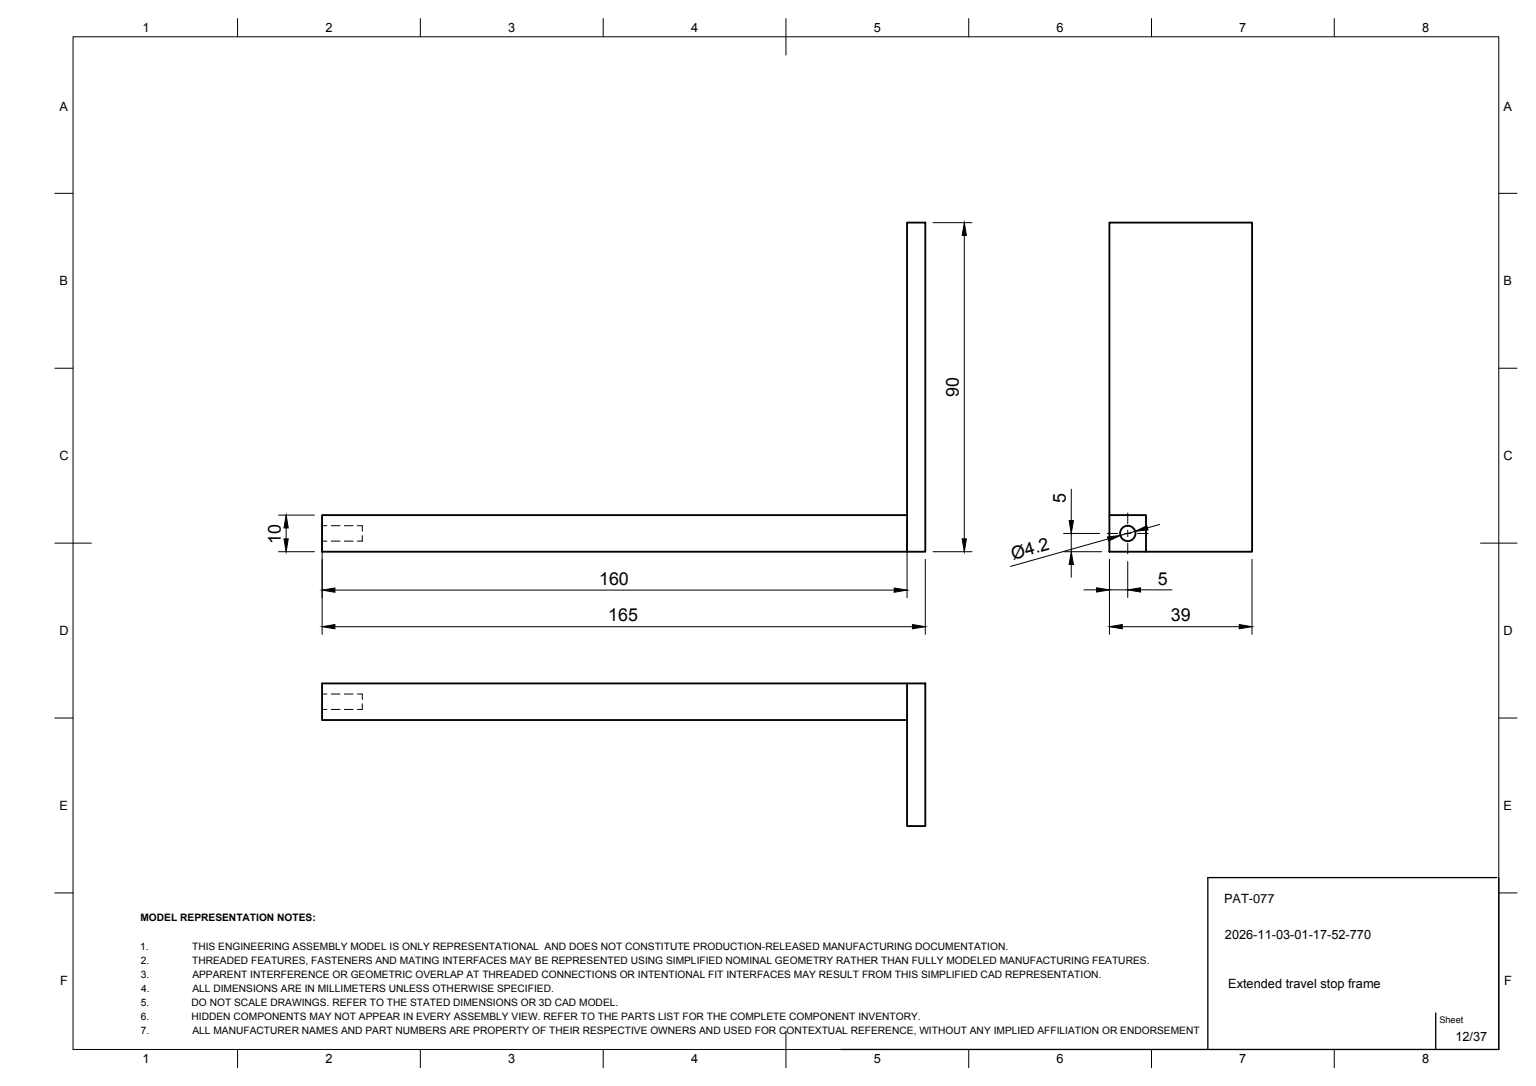
ISO-10303-21;
HEADER;
/* Generated by software containing ST-Developer
 * from STEP Tools, Inc. (www.steptools.com) 
 */

FILE_DESCRIPTION(
/* description */ ('Pallet stop with pneumatic fitting'),
/* implementation_level */ '2;1');

FILE_NAME(
/* name */ 'Extended travel stop frame.step',
/* time_stamp */ '2026-10-27T10:51:41-07:00',
/* author */ (''),
/* organization */ (''),
/* preprocessor_version */ 'ST-DEVELOPER v20.2',
/* originating_system */ 'Autodesk Translation Framework v15.17.0.0',
/* authorisation */ '');

FILE_SCHEMA (('AUTOMOTIVE_DESIGN { 1 0 10303 214 3 1 1 }'));
ENDSEC;

DATA;
#10=MECHANICAL_DESIGN_GEOMETRIC_PRESENTATION_REPRESENTATION('',(#364),#10265);
#300=SHAPE_REPRESENTATION_RELATIONSHIP('SRR','None',#10413,#332);
#332=ADVANCED_BREP_SHAPE_REPRESENTATION('',(#396),#10237);
#364=STYLED_ITEM('',(#10634),#396);
#396=MANIFOLD_SOLID_BREP('Body1',#5052);
#465=FACE_BOUND('',#1184,.T.);
#589=PLANE('',#5587);
#590=PLANE('',#5588);
#591=PLANE('',#5589);
#592=PLANE('',#5590);
#593=PLANE('',#5591);
#594=PLANE('',#5592);
#595=PLANE('',#5593);
#596=PLANE('',#5594);
#597=PLANE('',#5595);
#598=PLANE('',#5596);
#813=FACE_OUTER_BOUND('',#1173,.T.);
#814=FACE_OUTER_BOUND('',#1174,.T.);
#815=FACE_OUTER_BOUND('',#1175,.T.);
#816=FACE_OUTER_BOUND('',#1176,.T.);
#817=FACE_OUTER_BOUND('',#1177,.T.);
#818=FACE_OUTER_BOUND('',#1178,.T.);
#819=FACE_OUTER_BOUND('',#1179,.T.);
#820=FACE_OUTER_BOUND('',#1180,.T.);
#821=FACE_OUTER_BOUND('',#1181,.T.);
#822=FACE_OUTER_BOUND('',#1182,.T.);
#823=FACE_OUTER_BOUND('',#1183,.T.);
#1173=EDGE_LOOP('',(#3704,#3705,#3706,#3707));
#1174=EDGE_LOOP('',(#3708));
#1175=EDGE_LOOP('',(#3709,#3710,#3711,#3712,#3713,#3714));
#1176=EDGE_LOOP('',(#3715,#3716,#3717,#3718));
#1177=EDGE_LOOP('',(#3719,#3720,#3721,#3722));
#1178=EDGE_LOOP('',(#3723,#3724,#3725,#3726,#3727,#3728));
#1179=EDGE_LOOP('',(#3729,#3730,#3731,#3732,#3733,#3734));
#1180=EDGE_LOOP('',(#3735,#3736,#3737,#3738));
#1181=EDGE_LOOP('',(#3739,#3740,#3741,#3742));
#1182=EDGE_LOOP('',(#3743,#3744,#3745,#3746));
#1183=EDGE_LOOP('',(#3747,#3748,#3749,#3750));
#1184=EDGE_LOOP('',(#3751));
#1570=LINE('',#8908,#1905);
#1571=LINE('',#8914,#1906);
#1572=LINE('',#8916,#1907);
#1573=LINE('',#8918,#1908);
#1574=LINE('',#8920,#1909);
#1575=LINE('',#8922,#1910);
#1576=LINE('',#8923,#1911);
#1577=LINE('',#8926,#1912);
#1578=LINE('',#8928,#1913);
#1579=LINE('',#8929,#1914);
#1580=LINE('',#8932,#1915);
#1581=LINE('',#8933,#1916);
#1582=LINE('',#8937,#1917);
#1583=LINE('',#8939,#1918);
#1584=LINE('',#8940,#1919);
#1585=LINE('',#8941,#1920);
#1586=LINE('',#8944,#1921);
#1587=LINE('',#8945,#1922);
#1588=LINE('',#8946,#1923);
#1589=LINE('',#8949,#1924);
#1590=LINE('',#8950,#1925);
#1591=LINE('',#8952,#1926);
#1905=VECTOR('',#6477,0.21);
#1906=VECTOR('',#6484,1.);
#1907=VECTOR('',#6485,1.);
#1908=VECTOR('',#6486,1.);
#1909=VECTOR('',#6487,1.);
#1910=VECTOR('',#6488,1.);
#1911=VECTOR('',#6489,1.);
#1912=VECTOR('',#6492,1.);
#1913=VECTOR('',#6493,1.);
#1914=VECTOR('',#6494,1.);
#1915=VECTOR('',#6497,1.);
#1916=VECTOR('',#6498,1.);
#1917=VECTOR('',#6501,1.);
#1918=VECTOR('',#6502,1.);
#1919=VECTOR('',#6503,1.);
#1920=VECTOR('',#6504,1.);
#1921=VECTOR('',#6507,1.);
#1922=VECTOR('',#6508,1.);
#1923=VECTOR('',#6509,1.);
#1924=VECTOR('',#6512,1.);
#1925=VECTOR('',#6513,1.);
#1926=VECTOR('',#6516,1.);
#2226=CIRCLE('',#5585,0.21);
#2227=CIRCLE('',#5586,0.21);
#2505=VERTEX_POINT('',#8905);
#2506=VERTEX_POINT('',#8907);
#2507=VERTEX_POINT('',#8912);
#2508=VERTEX_POINT('',#8913);
#2509=VERTEX_POINT('',#8915);
#2510=VERTEX_POINT('',#8917);
#2511=VERTEX_POINT('',#8919);
#2512=VERTEX_POINT('',#8921);
#2513=VERTEX_POINT('',#8925);
#2514=VERTEX_POINT('',#8927);
#2515=VERTEX_POINT('',#8931);
#2516=VERTEX_POINT('',#8935);
#2517=VERTEX_POINT('',#8936);
#2518=VERTEX_POINT('',#8938);
#2519=VERTEX_POINT('',#8943);
#2520=VERTEX_POINT('',#8948);
#2951=EDGE_CURVE('',#2505,#2505,#2226,.T.);
#2952=EDGE_CURVE('',#2505,#2506,#1570,.T.);
#2953=EDGE_CURVE('',#2506,#2506,#2227,.T.);
#2954=EDGE_CURVE('',#2507,#2508,#1571,.T.);
#2955=EDGE_CURVE('',#2509,#2507,#1572,.T.);
#2956=EDGE_CURVE('',#2510,#2509,#1573,.T.);
#2957=EDGE_CURVE('',#2511,#2510,#1574,.T.);
#2958=EDGE_CURVE('',#2512,#2511,#1575,.T.);
#2959=EDGE_CURVE('',#2508,#2512,#1576,.T.);
#2960=EDGE_CURVE('',#2510,#2513,#1577,.T.);
#2961=EDGE_CURVE('',#2514,#2513,#1578,.T.);
#2962=EDGE_CURVE('',#2511,#2514,#1579,.T.);
#2963=EDGE_CURVE('',#2515,#2514,#1580,.T.);
#2964=EDGE_CURVE('',#2512,#2515,#1581,.T.);
#2965=EDGE_CURVE('',#2516,#2517,#1582,.T.);
#2966=EDGE_CURVE('',#2516,#2518,#1583,.T.);
#2967=EDGE_CURVE('',#2518,#2508,#1584,.T.);
#2968=EDGE_CURVE('',#2517,#2515,#1585,.T.);
#2969=EDGE_CURVE('',#2519,#2509,#1586,.T.);
#2970=EDGE_CURVE('',#2519,#2516,#1587,.T.);
#2971=EDGE_CURVE('',#2513,#2517,#1588,.T.);
#2972=EDGE_CURVE('',#2520,#2507,#1589,.T.);
#2973=EDGE_CURVE('',#2520,#2519,#1590,.T.);
#2974=EDGE_CURVE('',#2518,#2520,#1591,.T.);
#3704=ORIENTED_EDGE('',*,*,#2951,.F.);
#3705=ORIENTED_EDGE('',*,*,#2952,.T.);
#3706=ORIENTED_EDGE('',*,*,#2953,.T.);
#3707=ORIENTED_EDGE('',*,*,#2952,.F.);
#3708=ORIENTED_EDGE('',*,*,#2953,.F.);
#3709=ORIENTED_EDGE('',*,*,#2954,.F.);
#3710=ORIENTED_EDGE('',*,*,#2955,.F.);
#3711=ORIENTED_EDGE('',*,*,#2956,.F.);
#3712=ORIENTED_EDGE('',*,*,#2957,.F.);
#3713=ORIENTED_EDGE('',*,*,#2958,.F.);
#3714=ORIENTED_EDGE('',*,*,#2959,.F.);
#3715=ORIENTED_EDGE('',*,*,#2957,.T.);
#3716=ORIENTED_EDGE('',*,*,#2960,.T.);
#3717=ORIENTED_EDGE('',*,*,#2961,.F.);
#3718=ORIENTED_EDGE('',*,*,#2962,.F.);
#3719=ORIENTED_EDGE('',*,*,#2958,.T.);
#3720=ORIENTED_EDGE('',*,*,#2962,.T.);
#3721=ORIENTED_EDGE('',*,*,#2963,.F.);
#3722=ORIENTED_EDGE('',*,*,#2964,.F.);
#3723=ORIENTED_EDGE('',*,*,#2965,.F.);
#3724=ORIENTED_EDGE('',*,*,#2966,.T.);
#3725=ORIENTED_EDGE('',*,*,#2967,.T.);
#3726=ORIENTED_EDGE('',*,*,#2959,.T.);
#3727=ORIENTED_EDGE('',*,*,#2964,.T.);
#3728=ORIENTED_EDGE('',*,*,#2968,.F.);
#3729=ORIENTED_EDGE('',*,*,#2969,.F.);
#3730=ORIENTED_EDGE('',*,*,#2970,.T.);
#3731=ORIENTED_EDGE('',*,*,#2965,.T.);
#3732=ORIENTED_EDGE('',*,*,#2971,.F.);
#3733=ORIENTED_EDGE('',*,*,#2960,.F.);
#3734=ORIENTED_EDGE('',*,*,#2956,.T.);
#3735=ORIENTED_EDGE('',*,*,#2955,.T.);
#3736=ORIENTED_EDGE('',*,*,#2972,.F.);
#3737=ORIENTED_EDGE('',*,*,#2973,.T.);
#3738=ORIENTED_EDGE('',*,*,#2969,.T.);
#3739=ORIENTED_EDGE('',*,*,#2954,.T.);
#3740=ORIENTED_EDGE('',*,*,#2967,.F.);
#3741=ORIENTED_EDGE('',*,*,#2974,.T.);
#3742=ORIENTED_EDGE('',*,*,#2972,.T.);
#3743=ORIENTED_EDGE('',*,*,#2971,.T.);
#3744=ORIENTED_EDGE('',*,*,#2968,.T.);
#3745=ORIENTED_EDGE('',*,*,#2963,.T.);
#3746=ORIENTED_EDGE('',*,*,#2961,.T.);
#3747=ORIENTED_EDGE('',*,*,#2970,.F.);
#3748=ORIENTED_EDGE('',*,*,#2973,.F.);
#3749=ORIENTED_EDGE('',*,*,#2974,.F.);
#3750=ORIENTED_EDGE('',*,*,#2966,.F.);
#3751=ORIENTED_EDGE('',*,*,#2951,.T.);
#4654=CYLINDRICAL_SURFACE('',#5584,0.21);
#4808=ADVANCED_FACE('',(#813),#4654,.F.);
#4809=ADVANCED_FACE('',(#814),#589,.F.);
#4810=ADVANCED_FACE('',(#815),#590,.F.);
#4811=ADVANCED_FACE('',(#816),#591,.T.);
#4812=ADVANCED_FACE('',(#817),#592,.T.);
#4813=ADVANCED_FACE('',(#818),#593,.T.);
#4814=ADVANCED_FACE('',(#819),#594,.T.);
#4815=ADVANCED_FACE('',(#820),#595,.T.);
#4816=ADVANCED_FACE('',(#821),#596,.T.);
#4817=ADVANCED_FACE('',(#822),#597,.T.);
#4818=ADVANCED_FACE('',(#823,#465),#598,.F.);
#5052=CLOSED_SHELL('',(#4808,#4809,#4810,#4811,#4812,#4813,#4814,#4815,
#4816,#4817,#4818));
#5583=AXIS2_PLACEMENT_3D('',#8903,#6471,#6472);
#5584=AXIS2_PLACEMENT_3D('',#8904,#6473,#6474);
#5585=AXIS2_PLACEMENT_3D('',#8906,#6475,#6476);
#5586=AXIS2_PLACEMENT_3D('',#8909,#6478,#6479);
#5587=AXIS2_PLACEMENT_3D('',#8910,#6480,#6481);
#5588=AXIS2_PLACEMENT_3D('',#8911,#6482,#6483);
#5589=AXIS2_PLACEMENT_3D('',#8924,#6490,#6491);
#5590=AXIS2_PLACEMENT_3D('',#8930,#6495,#6496);
#5591=AXIS2_PLACEMENT_3D('',#8934,#6499,#6500);
#5592=AXIS2_PLACEMENT_3D('',#8942,#6505,#6506);
#5593=AXIS2_PLACEMENT_3D('',#8947,#6510,#6511);
#5594=AXIS2_PLACEMENT_3D('',#8951,#6514,#6515);
#5595=AXIS2_PLACEMENT_3D('',#8953,#6517,#6518);
#5596=AXIS2_PLACEMENT_3D('',#8954,#6519,#6520);
#6471=DIRECTION('axis',(0.,0.,1.));
#6472=DIRECTION('refdir',(1.,0.,0.));
#6473=DIRECTION('center_axis',(0.,0.,1.));
#6474=DIRECTION('ref_axis',(1.,0.,0.));
#6475=DIRECTION('center_axis',(0.,0.,1.));
#6476=DIRECTION('ref_axis',(1.,0.,0.));
#6477=DIRECTION('',(0.,0.,1.));
#6478=DIRECTION('center_axis',(0.,0.,1.));
#6479=DIRECTION('ref_axis',(1.,0.,0.));
#6480=DIRECTION('center_axis',(0.,0.,1.));
#6481=DIRECTION('ref_axis',(1.,0.,0.));
#6482=DIRECTION('center_axis',(0.,0.,1.));
#6483=DIRECTION('ref_axis',(1.,0.,0.));
#6484=DIRECTION('',(0.,-1.,0.));
#6485=DIRECTION('',(1.,0.,0.));
#6486=DIRECTION('',(0.,-1.,0.));
#6487=DIRECTION('',(-1.,0.,0.));
#6488=DIRECTION('',(0.,1.,0.));
#6489=DIRECTION('',(1.,0.,0.));
#6490=DIRECTION('center_axis',(0.,1.,0.));
#6491=DIRECTION('ref_axis',(-1.,0.,0.));
#6492=DIRECTION('',(0.,0.,1.));
#6493=DIRECTION('',(-1.,0.,0.));
#6494=DIRECTION('',(0.,0.,1.));
#6495=DIRECTION('center_axis',(1.,0.,0.));
#6496=DIRECTION('ref_axis',(0.,1.,0.));
#6497=DIRECTION('',(0.,1.,0.));
#6498=DIRECTION('',(0.,0.,1.));
#6499=DIRECTION('center_axis',(0.,-1.,0.));
#6500=DIRECTION('ref_axis',(1.,0.,0.));
#6501=DIRECTION('',(0.,0.,1.));
#6502=DIRECTION('',(1.,0.,0.));
#6503=DIRECTION('',(0.,0.,1.));
#6504=DIRECTION('',(1.,0.,0.));
#6505=DIRECTION('center_axis',(-1.,0.,0.));
#6506=DIRECTION('ref_axis',(0.,-1.,0.));
#6507=DIRECTION('',(0.,0.,1.));
#6508=DIRECTION('',(0.,-1.,0.));
#6509=DIRECTION('',(0.,-1.,0.));
#6510=DIRECTION('center_axis',(0.,1.,0.));
#6511=DIRECTION('ref_axis',(-1.,0.,0.));
#6512=DIRECTION('',(0.,0.,1.));
#6513=DIRECTION('',(-1.,0.,0.));
#6514=DIRECTION('center_axis',(1.,0.,0.));
#6515=DIRECTION('ref_axis',(0.,1.,0.));
#6516=DIRECTION('',(0.,1.,0.));
#6517=DIRECTION('center_axis',(0.,0.,1.));
#6518=DIRECTION('ref_axis',(1.,0.,0.));
#6519=DIRECTION('center_axis',(0.,0.,1.));
#6520=DIRECTION('ref_axis',(1.,0.,0.));
#8903=CARTESIAN_POINT('',(0.,0.,0.));
#8904=CARTESIAN_POINT('Origin',(-4.,-3.,-0.1));
#8905=CARTESIAN_POINT('',(-4.21,-3.,0.));
#8906=CARTESIAN_POINT('Origin',(-4.,-3.,0.));
#8907=CARTESIAN_POINT('',(-4.21,-3.,1.1));
#8908=CARTESIAN_POINT('',(-4.21,-3.,-0.1));
#8909=CARTESIAN_POINT('Origin',(-4.,-3.,1.1));
#8910=CARTESIAN_POINT('Origin',(-4.,-3.,1.1));
#8911=CARTESIAN_POINT('Origin',(0.,-1.55,16.));
#8912=CARTESIAN_POINT('',(-3.5,-2.5,16.));
#8913=CARTESIAN_POINT('',(-3.5,-3.5,16.));
#8914=CARTESIAN_POINT('',(-3.5,-2.525,16.));
#8915=CARTESIAN_POINT('',(-4.5,-2.5,16.));
#8916=CARTESIAN_POINT('',(-1.75,-2.5,16.));
#8917=CARTESIAN_POINT('',(-4.5,0.4,16.));
#8918=CARTESIAN_POINT('',(-4.5,0.4,16.));
#8919=CARTESIAN_POINT('',(4.5,0.4,16.));
#8920=CARTESIAN_POINT('',(4.5,0.4,16.));
#8921=CARTESIAN_POINT('',(4.5,-3.5,16.));
#8922=CARTESIAN_POINT('',(4.5,-3.5,16.));
#8923=CARTESIAN_POINT('',(-4.5,-3.5,16.));
#8924=CARTESIAN_POINT('Origin',(4.5,0.4,16.));
#8925=CARTESIAN_POINT('',(-4.5,0.4,16.5));
#8926=CARTESIAN_POINT('',(-4.5,0.4,16.));
#8927=CARTESIAN_POINT('',(4.5,0.4,16.5));
#8928=CARTESIAN_POINT('',(4.5,0.4,16.5));
#8929=CARTESIAN_POINT('',(4.5,0.4,16.));
#8930=CARTESIAN_POINT('Origin',(4.5,-3.5,16.));
#8931=CARTESIAN_POINT('',(4.5,-3.5,16.5));
#8932=CARTESIAN_POINT('',(4.5,-3.5,16.5));
#8933=CARTESIAN_POINT('',(4.5,-3.5,16.));
#8934=CARTESIAN_POINT('Origin',(-4.5,-3.5,0.));
#8935=CARTESIAN_POINT('',(-4.5,-3.5,0.));
#8936=CARTESIAN_POINT('',(-4.5,-3.5,16.5));
#8937=CARTESIAN_POINT('',(-4.5,-3.5,0.));
#8938=CARTESIAN_POINT('',(-3.5,-3.5,0.));
#8939=CARTESIAN_POINT('',(-4.5,-3.5,0.));
#8940=CARTESIAN_POINT('',(-3.5,-3.5,0.));
#8941=CARTESIAN_POINT('',(-4.5,-3.5,16.5));
#8942=CARTESIAN_POINT('Origin',(-4.5,-2.5,0.));
#8943=CARTESIAN_POINT('',(-4.5,-2.5,0.));
#8944=CARTESIAN_POINT('',(-4.5,-2.5,0.));
#8945=CARTESIAN_POINT('',(-4.5,-2.5,0.));
#8946=CARTESIAN_POINT('',(-4.5,0.4,16.5));
#8947=CARTESIAN_POINT('Origin',(-3.5,-2.5,0.));
#8948=CARTESIAN_POINT('',(-3.5,-2.5,0.));
#8949=CARTESIAN_POINT('',(-3.5,-2.5,0.));
#8950=CARTESIAN_POINT('',(-3.5,-2.5,0.));
#8951=CARTESIAN_POINT('Origin',(-3.5,-3.5,0.));
#8952=CARTESIAN_POINT('',(-3.5,-3.5,0.));
#8953=CARTESIAN_POINT('Origin',(-4.,-3.,16.5));
#8954=CARTESIAN_POINT('Origin',(-4.,-3.,0.));
#10199=UNCERTAINTY_MEASURE_WITH_UNIT(LENGTH_MEASURE(0.001),#10266,
'DISTANCE_ACCURACY_VALUE',
'Maximum model space distance between geometric entities at asserted c
onnectivities');
#10227=UNCERTAINTY_MEASURE_WITH_UNIT(LENGTH_MEASURE(0.001),#10266,
'DISTANCE_ACCURACY_VALUE',
'Maximum model space distance between geometric entities at asserted c
onnectivities');
#10237=(
GEOMETRIC_REPRESENTATION_CONTEXT(3)
GLOBAL_UNCERTAINTY_ASSIGNED_CONTEXT((#10199))
GLOBAL_UNIT_ASSIGNED_CONTEXT((#10266,#10268,#10269))
REPRESENTATION_CONTEXT('','3D')
);
#10265=(
GEOMETRIC_REPRESENTATION_CONTEXT(3)
GLOBAL_UNCERTAINTY_ASSIGNED_CONTEXT((#10227))
GLOBAL_UNIT_ASSIGNED_CONTEXT((#10266,#10268,#10269))
REPRESENTATION_CONTEXT('','3D')
);
#10266=(
LENGTH_UNIT()
NAMED_UNIT(*)
SI_UNIT(.CENTI.,.METRE.)
);
#10268=(
NAMED_UNIT(*)
PLANE_ANGLE_UNIT()
SI_UNIT($,.RADIAN.)
);
#10269=(
NAMED_UNIT(*)
SI_UNIT($,.STERADIAN.)
SOLID_ANGLE_UNIT()
);
#10279=SHAPE_DEFINITION_REPRESENTATION(#10316,#10413);
#10316=PRODUCT_DEFINITION_SHAPE('',$,#10451);
#10413=SHAPE_REPRESENTATION('',(#5583),#10237);
#10441=PRODUCT_DEFINITION_CONTEXT('part definition',#10554,'design');
#10451=PRODUCT_DEFINITION('Extended travel stop frame',
'Extended travel stop frame',#10488,#10441);
#10488=PRODUCT_DEFINITION_FORMATION('',$,#10565);
#10554=APPLICATION_CONTEXT(
'Core Data for Automotive Mechanical Design Process');
#10555=PRODUCT_CONTEXT('part definition',#10554,'mechanical');
#10565=PRODUCT('Extended travel stop frame',
'Extended travel stop frame','Extended travel stop frame',(#10555));
#10628=COLOUR_RGB('Dark Blue',0.08,0.2,0.34);
#10629=FILL_AREA_STYLE_COLOUR('',#10628);
#10630=FILL_AREA_STYLE('',(#10629));
#10631=SURFACE_STYLE_FILL_AREA(#10630);
#10632=SURFACE_SIDE_STYLE('',(#10631));
#10633=SURFACE_STYLE_USAGE(.BOTH.,#10632);
#10634=PRESENTATION_STYLE_ASSIGNMENT((#10633));
ENDSEC;
END-ISO-10303-21;
